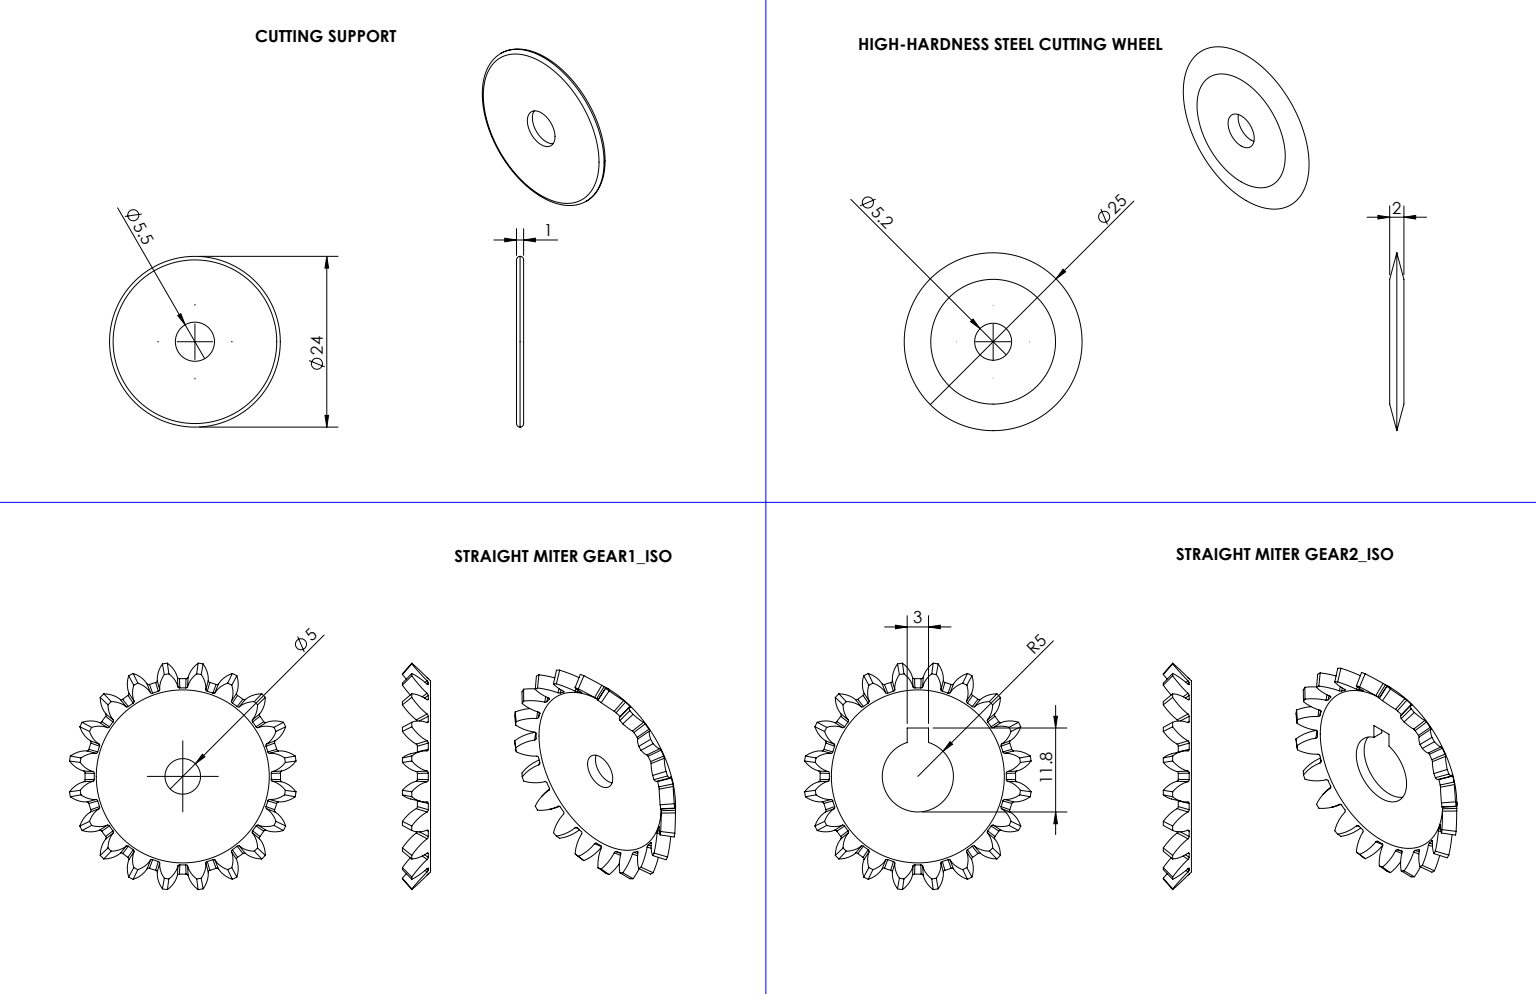
ISO-10303-21;
HEADER;
FILE_DESCRIPTION (('STEP AP214'),
    '1' );
FILE_NAME ('cutting support.step',
    '2026-09-24T10:15:42',
    ( '' ),
    ( '' ),
    'SwSTEP 2.0',
    'SolidWorks 2026',
    '' );
FILE_SCHEMA (( 'AUTOMOTIVE_DESIGN' ));
ENDSEC;

DATA;
#67=CYLINDRICAL_SURFACE ( 'NONE', #3011, 2.750000000000000000 ) ;
#82=ORIENTED_EDGE ( 'NONE', *, *, #18239, .T. ) ;
#114=CARTESIAN_POINT ( 'NONE',  ( 2.750000000000000000, 0.000000000000000000, 11.00000000000000000 ) ) ;
#202=VERTEX_POINT ( 'NONE', #18100 ) ;
#254=CIRCLE ( 'NONE', #4224, 11.50000000000000178 ) ;
#440=EDGE_CURVE ( 'NONE', #202, #1814, #17586, .T. ) ;
#596=ORIENTED_EDGE ( 'NONE', *, *, #12490, .T. ) ;
#650=CARTESIAN_POINT ( 'NONE',  ( 0.000000000000000000, 0.000000000000000000, 10.49999999999999822 ) ) ;
#728=TOROIDAL_SURFACE ( 'NONE', #7132, 11.50000000000000178, 0.5000000000000000000 ) ;
#868=ORIENTED_EDGE ( 'NONE', *, *, #18008, .F. ) ;
#874=CARTESIAN_POINT ( 'NONE',  ( 0.000000000000000000, 0.000000000000000000, 11.00000000000000000 ) ) ;
#942=DIRECTION ( 'NONE',  ( -0.000000000000000000, -0.000000000000000000, -1.000000000000000000 ) ) ;
#953=DIRECTION ( 'NONE',  ( 0.000000000000000000, -1.000000000000000000, 0.000000000000000000 ) ) ;
#985=SHAPE_DEFINITION_REPRESENTATION ( #14856, #9604 ) ;
#999=AXIS2_PLACEMENT_3D ( 'NONE', #650, #13915, #13738 ) ;
#1080=CARTESIAN_POINT ( 'NONE',  ( 2.750000000000000000, 0.000000000000000000, 10.00000000000000000 ) ) ;
#1170=CARTESIAN_POINT ( 'NONE',  ( 11.50000000000000178, 0.000000000000000000, 11.00000000000000000 ) ) ;
#1265=CARTESIAN_POINT ( 'NONE',  ( -11.50000000000000178, 1.438959988998140357E-15, 10.00000000000000000 ) ) ;
#1384=AXIS2_PLACEMENT_3D ( 'NONE', #11061, #7830, #17957 ) ;
#1422=ADVANCED_FACE ( 'NONE', ( #8943 ), #728, .T. ) ;
#1607=EDGE_CURVE ( 'NONE', #15230, #1814, #11495, .T. ) ;
#1639=DIRECTION ( 'NONE',  ( 0.000000000000000000, -1.000000000000000000, 0.000000000000000000 ) ) ;
#1683=DIRECTION ( 'NONE',  ( 0.000000000000000000, 0.000000000000000000, 1.000000000000000000 ) ) ;
#1684=AXIS2_PLACEMENT_3D ( 'NONE', #9479, #10822, #6338 ) ;
#1787=CARTESIAN_POINT ( 'NONE',  ( 0.000000000000000000, 0.000000000000000000, 10.50000000000000000 ) ) ;
#1806=EDGE_CURVE ( 'NONE', #14209, #13318, #2642, .T. ) ;
#1814=VERTEX_POINT ( 'NONE', #4011 ) ;
#1973=( NAMED_UNIT ( * ) SI_UNIT ( $, .STERADIAN. ) SOLID_ANGLE_UNIT ( ) );
#2030=AXIS2_PLACEMENT_3D ( 'NONE', #15716, #11248, #17249 ) ;
#2162=PRESENTATION_STYLE_ASSIGNMENT (( #3391 ) ) ;
#2242=SURFACE_SIDE_STYLE ('',( #3680 ) ) ;
#2330=SURFACE_STYLE_USAGE ( .BOTH. , #2593 ) ;
#2391=DIRECTION ( 'NONE',  ( 1.000000000000000000, 0.000000000000000000, 0.000000000000000000 ) ) ;
#2404=CYLINDRICAL_SURFACE ( 'NONE', #17854, 2.750000000000000000 ) ;
#2520=CARTESIAN_POINT ( 'NONE',  ( 0.000000000000000000, 0.000000000000000000, 10.49999999999999822 ) ) ;
#2558=VERTEX_POINT ( 'NONE', #10462 ) ;
#2593=SURFACE_SIDE_STYLE ('',( #6822 ) ) ;
#2624=( GEOMETRIC_REPRESENTATION_CONTEXT ( 3 ) GLOBAL_UNCERTAINTY_ASSIGNED_CONTEXT ( ( #11867 ) ) GLOBAL_UNIT_ASSIGNED_CONTEXT ( ( #18471, #18652, #13989 ) ) REPRESENTATION_CONTEXT ( 'NONE', 'WORKASPACE' ) );
#2642=CIRCLE ( 'NONE', #13341, 0.5000000000000004441 ) ;
#2653=DIRECTION ( 'NONE',  ( 0.000000000000000000, 0.000000000000000000, -1.000000000000000000 ) ) ;
#2787=VERTEX_POINT ( 'NONE', #1170 ) ;
#3011=AXIS2_PLACEMENT_3D ( 'NONE', #14683, #5788, #4368 ) ;
#3171=AXIS2_PLACEMENT_3D ( 'NONE', #13697, #4906, #10736 ) ;
#3391=SURFACE_STYLE_USAGE ( .BOTH. , #2242 ) ;
#3577=PRODUCT ( 'cutting support', 'cutting support', '', ( #15240 ) ) ;
#3581=( NAMED_UNIT ( * ) PLANE_ANGLE_UNIT ( ) SI_UNIT ( $, .RADIAN. ) );
#3680=SURFACE_STYLE_FILL_AREA ( #9229 ) ;
#3740=FACE_BOUND ( 'NONE', #18372, .T. ) ;
#3827=CARTESIAN_POINT ( 'NONE',  ( -11.50000000000000178, 1.408343819019456373E-15, 10.50000000000000000 ) ) ;
#3847=CARTESIAN_POINT ( 'NONE',  ( 0.000000000000000000, 0.000000000000000000, 10.50000000000000000 ) ) ;
#3872=ORIENTED_EDGE ( 'NONE', *, *, #13334, .F. ) ;
#4011=CARTESIAN_POINT ( 'NONE',  ( 2.750000000000000000, 0.000000000000000000, 11.00000000000000000 ) ) ;
#4088=FACE_OUTER_BOUND ( 'NONE', #13282, .T. ) ;
#4169=STYLED_ITEM ( 'NONE', ( #2162 ), #16154 ) ;
#4224=AXIS2_PLACEMENT_3D ( 'NONE', #12507, #6693, #13494 ) ;
#4268=VERTEX_POINT ( 'NONE', #14805 ) ;
#4270=ORIENTED_EDGE ( 'NONE', *, *, #1806, .F. ) ;
#4368=DIRECTION ( 'NONE',  ( 1.000000000000000000, 0.000000000000000000, 0.000000000000000000 ) ) ;
#4510=TOROIDAL_SURFACE ( 'NONE', #11532, 11.50000000000000178, 0.5000000000000000000 ) ;
#4713=CARTESIAN_POINT ( 'NONE',  ( 12.00000000000000178, 0.000000000000000000, 10.49999999999999822 ) ) ;
#4906=DIRECTION ( 'NONE',  ( 0.000000000000000000, 0.000000000000000000, 1.000000000000000000 ) ) ;
#5073=DIRECTION ( 'NONE',  ( -1.000000000000000000, 1.224646799147353454E-16, 0.000000000000000000 ) ) ;
#5094=APPLICATION_CONTEXT ( 'automotive_design' ) ;
#5131=CARTESIAN_POINT ( 'NONE',  ( 0.000000000000000000, 0.000000000000000000, 10.00000000000000000 ) ) ;
#5207=ADVANCED_FACE ( 'NONE', ( #3740, #6530 ), #5267, .T. ) ;
#5267=PLANE ( 'NONE',  #3171 ) ;
#5340=CIRCLE ( 'NONE', #16015, 2.750000000000000000 ) ;
#5382=( GEOMETRIC_REPRESENTATION_CONTEXT ( 3 ) GLOBAL_UNCERTAINTY_ASSIGNED_CONTEXT ( ( #7478 ) ) GLOBAL_UNIT_ASSIGNED_CONTEXT ( ( #15328, #3581, #16496 ) ) REPRESENTATION_CONTEXT ( 'NONE', 'WORKASPACE' ) );
#5437=EDGE_LOOP ( 'NONE', ( #14926, #11910, #8580, #82 ) ) ;
#5470=FILL_AREA_STYLE_COLOUR ( '', #7544 ) ;
#5534=CIRCLE ( 'NONE', #18667, 2.750000000000000000 ) ;
#5696=DIRECTION ( 'NONE',  ( 1.000000000000000000, 0.000000000000000000, 0.000000000000000000 ) ) ;
#5755=ORIENTED_EDGE ( 'NONE', *, *, #13094, .T. ) ;
#5788=DIRECTION ( 'NONE',  ( -0.000000000000000000, -0.000000000000000000, 1.000000000000000000 ) ) ;
#6238=PRODUCT_DEFINITION_FORMATION_WITH_SPECIFIED_SOURCE ( 'ANY', '', #3577, .NOT_KNOWN. ) ;
#6280=EDGE_LOOP ( 'NONE', ( #12272, #596, #10068, #14892 ) ) ;
#6338=DIRECTION ( 'NONE',  ( 1.000000000000000000, 0.000000000000000000, -0.000000000000000000 ) ) ;
#6346=DIRECTION ( 'NONE',  ( 1.224646799147353207E-16, 1.000000000000000000, -0.000000000000000000 ) ) ;
#6516=EDGE_CURVE ( 'NONE', #15230, #4268, #5534, .T. ) ;
#6530=FACE_OUTER_BOUND ( 'NONE', #12920, .T. ) ;
#6618=COLOUR_RGB ( '', 0.31764706, 0.68627451, 0.89019608) ;
#6631=EDGE_CURVE ( 'NONE', #4268, #202, #8228, .T. ) ;
#6641=EDGE_CURVE ( 'NONE', #14355, #14429, #16554, .T. ) ;
#6693=DIRECTION ( 'NONE',  ( 0.000000000000000000, 0.000000000000000000, 1.000000000000000000 ) ) ;
#6761=CIRCLE ( 'NONE', #14682, 11.50000000000000178 ) ;
#6822=SURFACE_STYLE_FILL_AREA ( #12642 ) ;
#6915=UNCERTAINTY_MEASURE_WITH_UNIT (LENGTH_MEASURE( 1.000000000000000082E-05 ), #15055, 'distance_accuracy_value', 'NONE');
#7002=DIRECTION ( 'NONE',  ( 1.000000000000000000, 0.000000000000000000, 0.000000000000000000 ) ) ;
#7111=ORIENTED_EDGE ( 'NONE', *, *, #1806, .T. ) ;
#7128=DIRECTION ( 'NONE',  ( 0.000000000000000000, 0.000000000000000000, 1.000000000000000000 ) ) ;
#7132=AXIS2_PLACEMENT_3D ( 'NONE', #1787, #1683, #13345 ) ;
#7193=CIRCLE ( 'NONE', #1384, 11.50000000000000178 ) ;
#7421=ADVANCED_FACE ( 'NONE', ( #14158 ), #10847, .T. ) ;
#7426=ADVANCED_FACE ( 'NONE', ( #18840 ), #2404, .F. ) ;
#7478=UNCERTAINTY_MEASURE_WITH_UNIT (LENGTH_MEASURE( 1.000000000000000082E-05 ), #15328, 'distance_accuracy_value', 'NONE');
#7484=CIRCLE ( 'NONE', #8695, 11.50000000000000178 ) ;
#7544=COLOUR_RGB ( '', 0.31764706, 0.68627451, 0.89019608) ;
#7546=ORIENTED_EDGE ( 'NONE', *, *, #13094, .F. ) ;
#7781=CARTESIAN_POINT ( 'NONE',  ( -11.50000000000000178, 1.408343819019456373E-15, 10.49999999999999822 ) ) ;
#7830=DIRECTION ( 'NONE',  ( -0.000000000000000000, -0.000000000000000000, -1.000000000000000000 ) ) ;
#7866=VECTOR ( 'NONE', #17605, 1000.000000000000000 ) ;
#8020=ORIENTED_EDGE ( 'NONE', *, *, #6641, .F. ) ;
#8228=LINE ( 'NONE', #17015, #9228 ) ;
#8256=DIRECTION ( 'NONE',  ( -0.000000000000000000, -0.000000000000000000, 1.000000000000000000 ) ) ;
#8318=CARTESIAN_POINT ( 'NONE',  ( 11.50000000000000178, 0.000000000000000000, 10.50000000000000000 ) ) ;
#8330=DIRECTION ( 'NONE',  ( 0.000000000000000000, 0.000000000000000000, 1.000000000000000000 ) ) ;
#8472=ORIENTED_EDGE ( 'NONE', *, *, #18239, .F. ) ;
#8580=ORIENTED_EDGE ( 'NONE', *, *, #1607, .T. ) ;
#8695=AXIS2_PLACEMENT_3D ( 'NONE', #874, #8330, #2391 ) ;
#8806=EDGE_LOOP ( 'NONE', ( #15947, #7111, #15982, #8020 ) ) ;
#8943=FACE_OUTER_BOUND ( 'NONE', #8806, .T. ) ;
#9107=CARTESIAN_POINT ( 'NONE',  ( 11.50000000000000178, 0.000000000000000000, 10.00000000000000000 ) ) ;
#9183=DIRECTION ( 'NONE',  ( 1.000000000000000000, 0.000000000000000000, 0.000000000000000000 ) ) ;
#9228=VECTOR ( 'NONE', #15478, 1000.000000000000000 ) ;
#9229=FILL_AREA_STYLE ('',( #10671 ) ) ;
#9428=ORIENTED_EDGE ( 'NONE', *, *, #1607, .F. ) ;
#9429=EDGE_CURVE ( 'NONE', #14429, #2787, #18457, .T. ) ;
#9479=CARTESIAN_POINT ( 'NONE',  ( 0.000000000000000000, 0.000000000000000000, 10.00000000000000000 ) ) ;
#9525=ADVANCED_FACE ( 'NONE', ( #10728, #13961 ), #13778, .F. ) ;
#9544=AXIS2_PLACEMENT_3D ( 'NONE', #5131, #10973, #16794 ) ;
#9578=CARTESIAN_POINT ( 'NONE',  ( 0.000000000000000000, 0.000000000000000000, 11.00000000000000000 ) ) ;
#9604=SHAPE_REPRESENTATION ( 'cutting support', ( #2030 ), #5382 ) ;
#9655=DIRECTION ( 'NONE',  ( 1.224646799147353207E-16, 1.000000000000000000, -0.000000000000000000 ) ) ;
#9677=DIRECTION ( 'NONE',  ( 1.000000000000000000, 0.000000000000000000, 0.000000000000000000 ) ) ;
#9730=DIRECTION ( 'NONE',  ( 1.000000000000000000, 0.000000000000000000, 0.000000000000000000 ) ) ;
#9910=CARTESIAN_POINT ( 'NONE',  ( 0.000000000000000000, 0.000000000000000000, 10.49999999999999822 ) ) ;
#9943=ORIENTED_EDGE ( 'NONE', *, *, #18008, .T. ) ;
#10068=ORIENTED_EDGE ( 'NONE', *, *, #14338, .F. ) ;
#10149=EDGE_LOOP ( 'NONE', ( #18765, #11519, #17077, #9428 ) ) ;
#10439=AXIS2_PLACEMENT_3D ( 'NONE', #8318, #953, #2653 ) ;
#10462=CARTESIAN_POINT ( 'NONE',  ( -11.50000000000000178, 1.438959988998140357E-15, 11.00000000000000000 ) ) ;
#10602=ADVANCED_FACE ( 'NONE', ( #4088 ), #18726, .T. ) ;
#10671=FILL_AREA_STYLE_COLOUR ( '', #6618 ) ;
#10728=FACE_BOUND ( 'NONE', #12265, .T. ) ;
#10736=DIRECTION ( 'NONE',  ( 1.000000000000000000, 0.000000000000000000, -0.000000000000000000 ) ) ;
#10782=EDGE_CURVE ( 'NONE', #4268, #15230, #12891, .T. ) ;
#10787=CIRCLE ( 'NONE', #999, 12.00000000000000178 ) ;
#10822=DIRECTION ( 'NONE',  ( 0.000000000000000000, 0.000000000000000000, 1.000000000000000000 ) ) ;
#10847=TOROIDAL_SURFACE ( 'NONE', #15395, 11.50000000000000178, 0.5000000000000000000 ) ;
#10849=EDGE_CURVE ( 'NONE', #13318, #14429, #10787, .T. ) ;
#10881=DIRECTION ( 'NONE',  ( -0.000000000000000000, -0.000000000000000000, -1.000000000000000000 ) ) ;
#10915=( GEOMETRIC_REPRESENTATION_CONTEXT ( 3 ) GLOBAL_UNCERTAINTY_ASSIGNED_CONTEXT ( ( #6915 ) ) GLOBAL_UNIT_ASSIGNED_CONTEXT ( ( #15055, #13996, #1973 ) ) REPRESENTATION_CONTEXT ( 'NONE', 'WORKASPACE' ) );
#10973=DIRECTION ( 'NONE',  ( -0.000000000000000000, -0.000000000000000000, 1.000000000000000000 ) ) ;
#11049=CIRCLE ( 'NONE', #16835, 0.5000000000000004441 ) ;
#11061=CARTESIAN_POINT ( 'NONE',  ( 0.000000000000000000, 0.000000000000000000, 10.00000000000000000 ) ) ;
#11120=CARTESIAN_POINT ( 'NONE',  ( 0.000000000000000000, 0.000000000000000000, 11.00000000000000000 ) ) ;
#11248=DIRECTION ( 'NONE',  ( 0.000000000000000000, 0.000000000000000000, 1.000000000000000000 ) ) ;
#11317=PRESENTATION_STYLE_ASSIGNMENT (( #2330 ) ) ;
#11408=SHAPE_REPRESENTATION_RELATIONSHIP ( 'NONE' , 'NONE' ,  #9604, #16761 ) ;
#11495=LINE ( 'NONE', #114, #7866 ) ;
#11519=ORIENTED_EDGE ( 'NONE', *, *, #6631, .T. ) ;
#11532=AXIS2_PLACEMENT_3D ( 'NONE', #2520, #7128, #14012 ) ;
#11548=DIRECTION ( 'NONE',  ( 0.000000000000000000, 0.000000000000000000, 1.000000000000000000 ) ) ;
#11867=UNCERTAINTY_MEASURE_WITH_UNIT (LENGTH_MEASURE( 1.000000000000000082E-05 ), #18471, 'distance_accuracy_value', 'NONE');
#11910=ORIENTED_EDGE ( 'NONE', *, *, #6516, .F. ) ;
#11970=CARTESIAN_POINT ( 'NONE',  ( 11.50000000000000178, 0.000000000000000000, 10.49999999999999822 ) ) ;
#12007=ORIENTED_EDGE ( 'NONE', *, *, #9429, .T. ) ;
#12246=ORIENTED_EDGE ( 'NONE', *, *, #6516, .T. ) ;
#12257=CIRCLE ( 'NONE', #16536, 12.00000000000000178 ) ;
#12265=EDGE_LOOP ( 'NONE', ( #12246, #16113 ) ) ;
#12272=ORIENTED_EDGE ( 'NONE', *, *, #10849, .F. ) ;
#12418=STYLED_ITEM ( 'NONE', ( #11317 ), #16761 ) ;
#12490=EDGE_CURVE ( 'NONE', #13318, #2558, #11049, .T. ) ;
#12507=CARTESIAN_POINT ( 'NONE',  ( 0.000000000000000000, 0.000000000000000000, 11.00000000000000000 ) ) ;
#12642=FILL_AREA_STYLE ('',( #5470 ) ) ;
#12660=AXIS2_PLACEMENT_3D ( 'NONE', #11970, #1639, #17507 ) ;
#12872=CARTESIAN_POINT ( 'NONE',  ( 0.000000000000000000, 0.000000000000000000, 10.00000000000000000 ) ) ;
#12891=CIRCLE ( 'NONE', #9544, 2.750000000000000000 ) ;
#12920=EDGE_LOOP ( 'NONE', ( #18592, #9943 ) ) ;
#12989=CARTESIAN_POINT ( 'NONE',  ( 0.000000000000000000, 0.000000000000000000, 11.00000000000000000 ) ) ;
#13094=EDGE_CURVE ( 'NONE', #14429, #13318, #12257, .T. ) ;
#13190=DIRECTION ( 'NONE',  ( -0.000000000000000000, -0.000000000000000000, 1.000000000000000000 ) ) ;
#13282=EDGE_LOOP ( 'NONE', ( #18212, #7546, #12007, #868 ) ) ;
#13318=VERTEX_POINT ( 'NONE', #18423 ) ;
#13334=EDGE_CURVE ( 'NONE', #14355, #14209, #6761, .T. ) ;
#13341=AXIS2_PLACEMENT_3D ( 'NONE', #3827, #9655, #5073 ) ;
#13345=DIRECTION ( 'NONE',  ( 1.000000000000000000, 0.000000000000000000, 0.000000000000000000 ) ) ;
#13470=DIRECTION ( 'NONE',  ( -0.000000000000000000, -0.000000000000000000, 1.000000000000000000 ) ) ;
#13494=DIRECTION ( 'NONE',  ( 1.000000000000000000, 0.000000000000000000, 0.000000000000000000 ) ) ;
#13636=MECHANICAL_DESIGN_GEOMETRIC_PRESENTATION_REPRESENTATION('',(#12418),#2624);
#13648=MECHANICAL_DESIGN_GEOMETRIC_PRESENTATION_REPRESENTATION('',(#4169),#10915);
#13697=CARTESIAN_POINT ( 'NONE',  ( 0.000000000000000000, 0.000000000000000000, 11.00000000000000000 ) ) ;
#13738=DIRECTION ( 'NONE',  ( 1.000000000000000000, 0.000000000000000000, 0.000000000000000000 ) ) ;
#13778=PLANE ( 'NONE',  #1684 ) ;
#13809=ADVANCED_FACE ( 'NONE', ( #16976 ), #4510, .T. ) ;
#13814=ORIENTED_EDGE ( 'NONE', *, *, #13334, .T. ) ;
#13915=DIRECTION ( 'NONE',  ( -0.000000000000000000, -0.000000000000000000, -1.000000000000000000 ) ) ;
#13961=FACE_OUTER_BOUND ( 'NONE', #16979, .T. ) ;
#13989=( NAMED_UNIT ( * ) SI_UNIT ( $, .STERADIAN. ) SOLID_ANGLE_UNIT ( ) );
#13996=( NAMED_UNIT ( * ) PLANE_ANGLE_UNIT ( ) SI_UNIT ( $, .RADIAN. ) );
#14012=DIRECTION ( 'NONE',  ( 1.000000000000000000, 0.000000000000000000, 0.000000000000000000 ) ) ;
#14158=FACE_OUTER_BOUND ( 'NONE', #17726, .T. ) ;
#14209=VERTEX_POINT ( 'NONE', #1265 ) ;
#14338=EDGE_CURVE ( 'NONE', #2787, #2558, #254, .T. ) ;
#14355=VERTEX_POINT ( 'NONE', #9107 ) ;
#14429=VERTEX_POINT ( 'NONE', #4713 ) ;
#14628=CARTESIAN_POINT ( 'NONE',  ( 0.000000000000000000, 0.000000000000000000, 10.00000000000000000 ) ) ;
#14682=AXIS2_PLACEMENT_3D ( 'NONE', #12872, #942, #5696 ) ;
#14683=CARTESIAN_POINT ( 'NONE',  ( 0.000000000000000000, 0.000000000000000000, 11.00000000000000000 ) ) ;
#14805=CARTESIAN_POINT ( 'NONE',  ( -2.750000000000000000, 3.367778697655221012E-16, 10.00000000000000000 ) ) ;
#14856=PRODUCT_DEFINITION_SHAPE ( 'NONE', 'NONE',  #15021 ) ;
#14868=CLOSED_SHELL ( 'NONE', ( #7426, #1422, #13809, #5207, #9525, #10602, #7421, #17437 ) ) ;
#14892=ORIENTED_EDGE ( 'NONE', *, *, #9429, .F. ) ;
#14906=DIRECTION ( 'NONE',  ( 1.000000000000000000, 0.000000000000000000, 0.000000000000000000 ) ) ;
#14926=ORIENTED_EDGE ( 'NONE', *, *, #6631, .F. ) ;
#15021=PRODUCT_DEFINITION ( 'UNKNOWN', '', #6238, #16519 ) ;
#15027=DIRECTION ( 'NONE',  ( -1.000000000000000000, 1.224646799147353454E-16, 0.000000000000000000 ) ) ;
#15055=( LENGTH_UNIT ( ) NAMED_UNIT ( * ) SI_UNIT ( .MILLI., .METRE. ) );
#15151=AXIS2_PLACEMENT_3D ( 'NONE', #9578, #15409, #18456 ) ;
#15230=VERTEX_POINT ( 'NONE', #1080 ) ;
#15240=PRODUCT_CONTEXT ( 'NONE', #5094, 'mechanical' ) ;
#15261=DIRECTION ( 'NONE',  ( 1.000000000000000000, 0.000000000000000000, 0.000000000000000000 ) ) ;
#15328=( LENGTH_UNIT ( ) NAMED_UNIT ( * ) SI_UNIT ( .MILLI., .METRE. ) );
#15395=AXIS2_PLACEMENT_3D ( 'NONE', #3847, #15781, #9677 ) ;
#15409=DIRECTION ( 'NONE',  ( -0.000000000000000000, -0.000000000000000000, 1.000000000000000000 ) ) ;
#15478=DIRECTION ( 'NONE',  ( -0.000000000000000000, -0.000000000000000000, 1.000000000000000000 ) ) ;
#15716=CARTESIAN_POINT ( 'NONE',  ( 0.000000000000000000, 0.000000000000000000, 0.000000000000000000 ) ) ;
#15781=DIRECTION ( 'NONE',  ( 0.000000000000000000, 0.000000000000000000, 1.000000000000000000 ) ) ;
#15947=ORIENTED_EDGE ( 'NONE', *, *, #18806, .F. ) ;
#15982=ORIENTED_EDGE ( 'NONE', *, *, #10849, .T. ) ;
#16015=AXIS2_PLACEMENT_3D ( 'NONE', #12989, #13470, #14906 ) ;
#16113=ORIENTED_EDGE ( 'NONE', *, *, #10782, .T. ) ;
#16154=MANIFOLD_SOLID_BREP ( 'M5 Clearance Hole1', #14868 ) ;
#16181=ORIENTED_EDGE ( 'NONE', *, *, #440, .F. ) ;
#16325=FACE_OUTER_BOUND ( 'NONE', #5437, .T. ) ;
#16496=( NAMED_UNIT ( * ) SI_UNIT ( $, .STERADIAN. ) SOLID_ANGLE_UNIT ( ) );
#16519=PRODUCT_DEFINITION_CONTEXT ( 'detailed design', #17423, 'design' ) ;
#16536=AXIS2_PLACEMENT_3D ( 'NONE', #16791, #10881, #15261 ) ;
#16554=CIRCLE ( 'NONE', #10439, 0.5000000000000004441 ) ;
#16761=ADVANCED_BREP_SHAPE_REPRESENTATION ( '', ( #16154, #2030 ), #5382 ) ;
#16791=CARTESIAN_POINT ( 'NONE',  ( 0.000000000000000000, 0.000000000000000000, 10.49999999999999822 ) ) ;
#16794=DIRECTION ( 'NONE',  ( 1.000000000000000000, 0.000000000000000000, 0.000000000000000000 ) ) ;
#16835=AXIS2_PLACEMENT_3D ( 'NONE', #7781, #6346, #15027 ) ;
#16976=FACE_OUTER_BOUND ( 'NONE', #6280, .T. ) ;
#16979=EDGE_LOOP ( 'NONE', ( #13814, #18095 ) ) ;
#17015=CARTESIAN_POINT ( 'NONE',  ( -2.750000000000000000, 3.367778697655221012E-16, 11.00000000000000000 ) ) ;
#17077=ORIENTED_EDGE ( 'NONE', *, *, #440, .T. ) ;
#17249=DIRECTION ( 'NONE',  ( 1.000000000000000000, 0.000000000000000000, 0.000000000000000000 ) ) ;
#17262=ORIENTED_EDGE ( 'NONE', *, *, #6641, .T. ) ;
#17423=APPLICATION_CONTEXT ( 'automotive_design' ) ;
#17437=ADVANCED_FACE ( 'NONE', ( #16325 ), #67, .F. ) ;
#17507=DIRECTION ( 'NONE',  ( 0.000000000000000000, 0.000000000000000000, -1.000000000000000000 ) ) ;
#17586=CIRCLE ( 'NONE', #15151, 2.750000000000000000 ) ;
#17605=DIRECTION ( 'NONE',  ( -0.000000000000000000, -0.000000000000000000, 1.000000000000000000 ) ) ;
#17726=EDGE_LOOP ( 'NONE', ( #4270, #3872, #17262, #5755 ) ) ;
#17837=AXIS2_PLACEMENT_3D ( 'NONE', #9910, #11548, #9730 ) ;
#17854=AXIS2_PLACEMENT_3D ( 'NONE', #11120, #8256, #7002 ) ;
#17957=DIRECTION ( 'NONE',  ( 1.000000000000000000, 0.000000000000000000, 0.000000000000000000 ) ) ;
#18008=EDGE_CURVE ( 'NONE', #2558, #2787, #7484, .T. ) ;
#18095=ORIENTED_EDGE ( 'NONE', *, *, #18806, .T. ) ;
#18100=CARTESIAN_POINT ( 'NONE',  ( -2.750000000000000000, 3.367778697655221012E-16, 11.00000000000000000 ) ) ;
#18212=ORIENTED_EDGE ( 'NONE', *, *, #12490, .F. ) ;
#18239=EDGE_CURVE ( 'NONE', #1814, #202, #5340, .T. ) ;
#18372=EDGE_LOOP ( 'NONE', ( #8472, #16181 ) ) ;
#18423=CARTESIAN_POINT ( 'NONE',  ( -12.00000000000000178, 1.469576158976824144E-15, 10.49999999999999822 ) ) ;
#18456=DIRECTION ( 'NONE',  ( 1.000000000000000000, 0.000000000000000000, 0.000000000000000000 ) ) ;
#18457=CIRCLE ( 'NONE', #12660, 0.5000000000000004441 ) ;
#18471=( LENGTH_UNIT ( ) NAMED_UNIT ( * ) SI_UNIT ( .MILLI., .METRE. ) );
#18592=ORIENTED_EDGE ( 'NONE', *, *, #14338, .T. ) ;
#18652=( NAMED_UNIT ( * ) PLANE_ANGLE_UNIT ( ) SI_UNIT ( $, .RADIAN. ) );
#18667=AXIS2_PLACEMENT_3D ( 'NONE', #14628, #13190, #9183 ) ;
#18726=TOROIDAL_SURFACE ( 'NONE', #17837, 11.50000000000000178, 0.5000000000000000000 ) ;
#18765=ORIENTED_EDGE ( 'NONE', *, *, #10782, .F. ) ;
#18806=EDGE_CURVE ( 'NONE', #14209, #14355, #7193, .T. ) ;
#18840=FACE_OUTER_BOUND ( 'NONE', #10149, .T. ) ;
ENDSEC;
END-ISO-10303-21;
